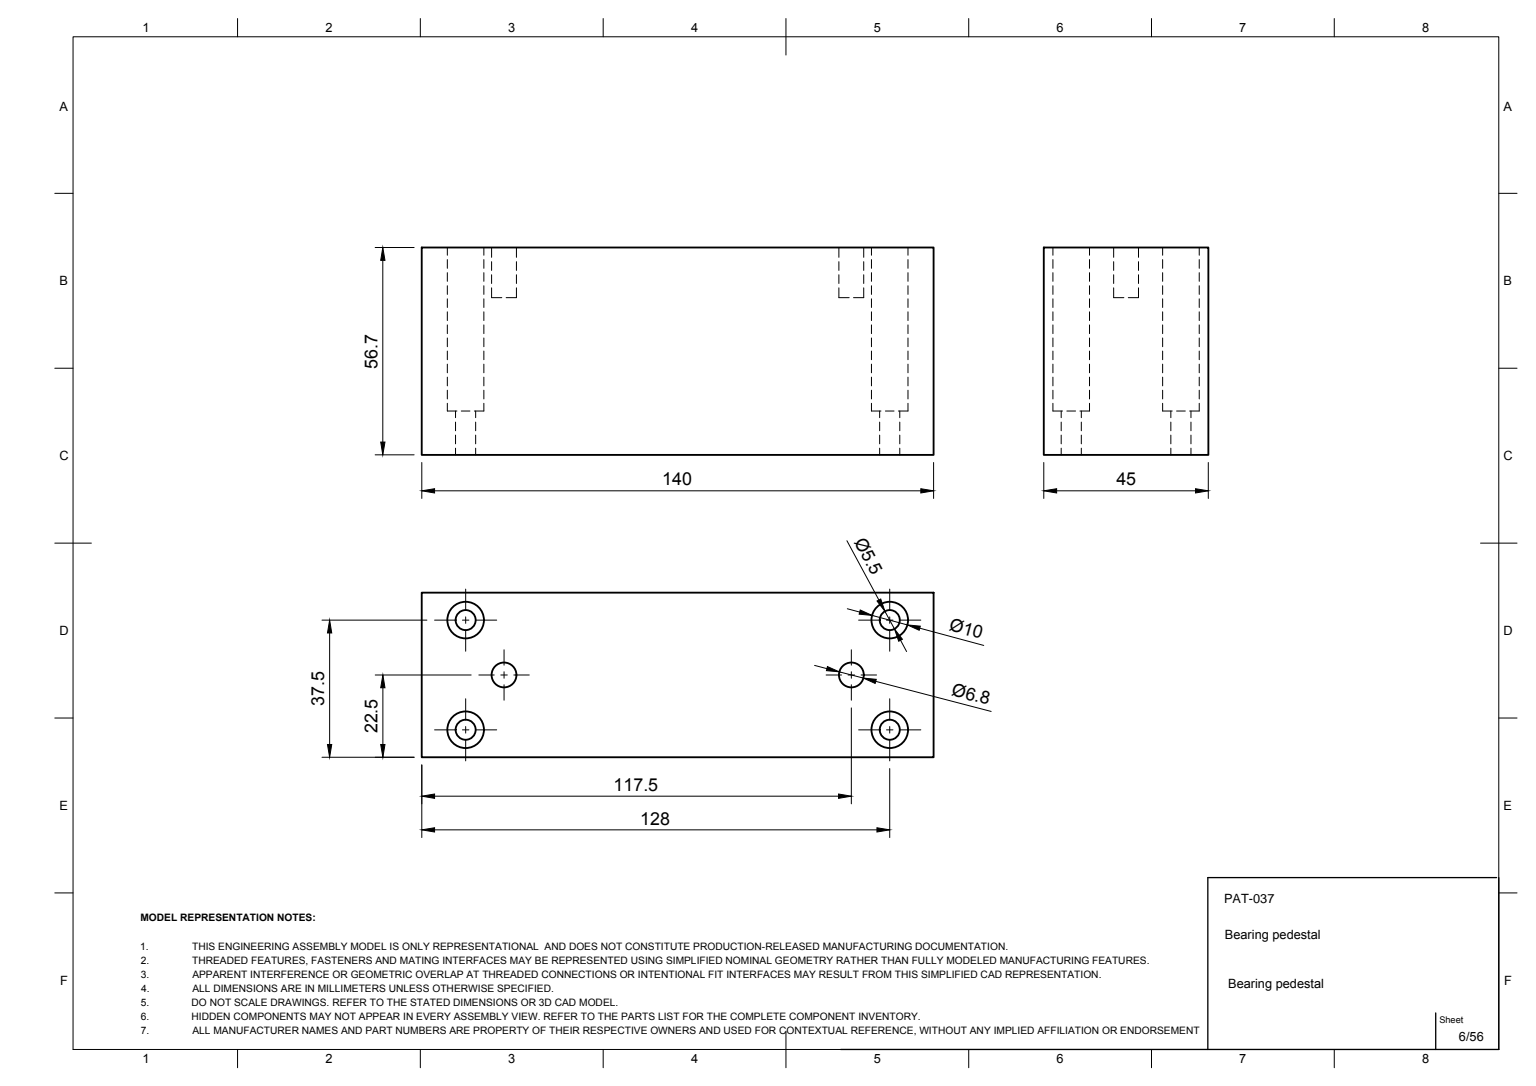
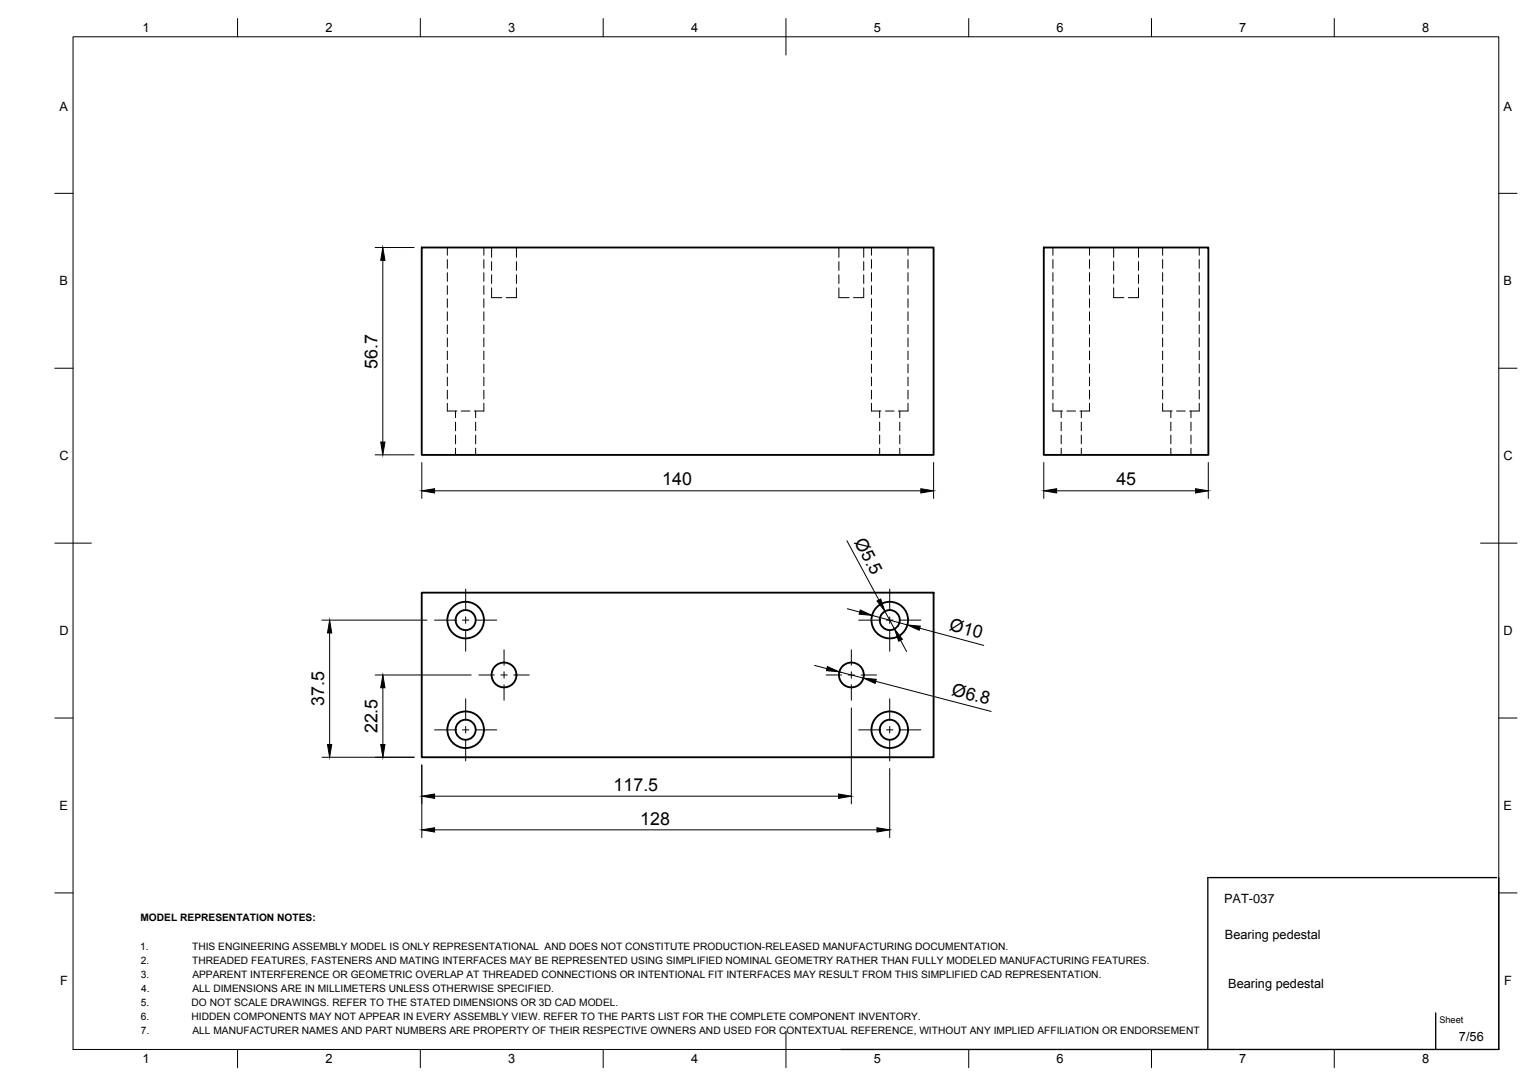
ISO-10303-21;
HEADER;
/* Generated by software containing ST-Developer
 * from STEP Tools, Inc. (www.steptools.com) 
 */

FILE_DESCRIPTION(
/* description */ ('Flywheel Crank-Slider'),
/* implementation_level */ '2;1');

FILE_NAME(
/* name */ 'Bearing pedestal.step',
/* time_stamp */ '2026-10-28T03:23:13-07:00',
/* author */ (''),
/* organization */ (''),
/* preprocessor_version */ 'ST-DEVELOPER v20.2',
/* originating_system */ 'Autodesk Translation Framework v15.17.0.0',
/* authorisation */ '');

FILE_SCHEMA (('AUTOMOTIVE_DESIGN { 1 0 10303 214 3 1 1 }'));
ENDSEC;

DATA;
#10=MECHANICAL_DESIGN_GEOMETRIC_PRESENTATION_REPRESENTATION('',(#669),#17322);
#565=SHAPE_REPRESENTATION_RELATIONSHIP('SRR','None',#17561,#617);
#617=ADVANCED_BREP_SHAPE_REPRESENTATION('',(#730),#17265);
#669=STYLED_ITEM('',(#17931),#730);
#730=MANIFOLD_SOLID_BREP('Body1',#9047);
#809=FACE_BOUND('',#1903,.T.);
#810=FACE_BOUND('',#1906,.T.);
#811=FACE_BOUND('',#1909,.T.);
#812=FACE_BOUND('',#1912,.T.);
#813=FACE_BOUND('',#1922,.T.);
#814=FACE_BOUND('',#1923,.T.);
#815=FACE_BOUND('',#1924,.T.);
#816=FACE_BOUND('',#1925,.T.);
#817=FACE_BOUND('',#1926,.T.);
#818=FACE_BOUND('',#1927,.T.);
#819=FACE_BOUND('',#1929,.T.);
#820=FACE_BOUND('',#1930,.T.);
#821=FACE_BOUND('',#1931,.T.);
#822=FACE_BOUND('',#1932,.T.);
#1017=PLANE('',#9734);
#1018=PLANE('',#9738);
#1019=PLANE('',#9742);
#1020=PLANE('',#9747);
#1021=PLANE('',#9752);
#1022=PLANE('',#9757);
#1023=PLANE('',#9767);
#1024=PLANE('',#9768);
#1025=PLANE('',#9769);
#1026=PLANE('',#9770);
#1027=PLANE('',#9771);
#1028=PLANE('',#9772);
#1338=FACE_OUTER_BOUND('',#1897,.T.);
#1339=FACE_OUTER_BOUND('',#1898,.T.);
#1340=FACE_OUTER_BOUND('',#1899,.T.);
#1341=FACE_OUTER_BOUND('',#1900,.T.);
#1342=FACE_OUTER_BOUND('',#1901,.T.);
#1343=FACE_OUTER_BOUND('',#1902,.T.);
#1344=FACE_OUTER_BOUND('',#1904,.T.);
#1345=FACE_OUTER_BOUND('',#1905,.T.);
#1346=FACE_OUTER_BOUND('',#1907,.T.);
#1347=FACE_OUTER_BOUND('',#1908,.T.);
#1348=FACE_OUTER_BOUND('',#1910,.T.);
#1349=FACE_OUTER_BOUND('',#1911,.T.);
#1350=FACE_OUTER_BOUND('',#1913,.T.);
#1351=FACE_OUTER_BOUND('',#1914,.T.);
#1352=FACE_OUTER_BOUND('',#1915,.T.);
#1353=FACE_OUTER_BOUND('',#1916,.T.);
#1354=FACE_OUTER_BOUND('',#1917,.T.);
#1355=FACE_OUTER_BOUND('',#1918,.T.);
#1356=FACE_OUTER_BOUND('',#1919,.T.);
#1357=FACE_OUTER_BOUND('',#1920,.T.);
#1358=FACE_OUTER_BOUND('',#1921,.T.);
#1359=FACE_OUTER_BOUND('',#1928,.T.);
#1897=EDGE_LOOP('',(#6218,#6219,#6220,#6221));
#1898=EDGE_LOOP('',(#6222));
#1899=EDGE_LOOP('',(#6223,#6224,#6225,#6226));
#1900=EDGE_LOOP('',(#6227));
#1901=EDGE_LOOP('',(#6228,#6229,#6230,#6231));
#1902=EDGE_LOOP('',(#6232));
#1903=EDGE_LOOP('',(#6233));
#1904=EDGE_LOOP('',(#6234,#6235,#6236,#6237));
#1905=EDGE_LOOP('',(#6238));
#1906=EDGE_LOOP('',(#6239));
#1907=EDGE_LOOP('',(#6240,#6241,#6242,#6243));
#1908=EDGE_LOOP('',(#6244));
#1909=EDGE_LOOP('',(#6245));
#1910=EDGE_LOOP('',(#6246,#6247,#6248,#6249));
#1911=EDGE_LOOP('',(#6250));
#1912=EDGE_LOOP('',(#6251));
#1913=EDGE_LOOP('',(#6252,#6253,#6254,#6255));
#1914=EDGE_LOOP('',(#6256,#6257,#6258,#6259));
#1915=EDGE_LOOP('',(#6260,#6261,#6262,#6263));
#1916=EDGE_LOOP('',(#6264,#6265,#6266,#6267));
#1917=EDGE_LOOP('',(#6268,#6269,#6270,#6271));
#1918=EDGE_LOOP('',(#6272,#6273,#6274,#6275));
#1919=EDGE_LOOP('',(#6276,#6277,#6278,#6279));
#1920=EDGE_LOOP('',(#6280,#6281,#6282,#6283));
#1921=EDGE_LOOP('',(#6284,#6285,#6286,#6287));
#1922=EDGE_LOOP('',(#6288));
#1923=EDGE_LOOP('',(#6289));
#1924=EDGE_LOOP('',(#6290));
#1925=EDGE_LOOP('',(#6291));
#1926=EDGE_LOOP('',(#6292));
#1927=EDGE_LOOP('',(#6293));
#1928=EDGE_LOOP('',(#6294,#6295,#6296,#6297));
#1929=EDGE_LOOP('',(#6298));
#1930=EDGE_LOOP('',(#6299));
#1931=EDGE_LOOP('',(#6300));
#1932=EDGE_LOOP('',(#6301));
#2640=LINE('',#13837,#3251);
#2641=LINE('',#13844,#3252);
#2642=LINE('',#13851,#3253);
#2643=LINE('',#13860,#3254);
#2644=LINE('',#13869,#3255);
#2645=LINE('',#13878,#3256);
#2646=LINE('',#13886,#3257);
#2647=LINE('',#13890,#3258);
#2648=LINE('',#13894,#3259);
#2649=LINE('',#13898,#3260);
#2650=LINE('',#13902,#3261);
#2651=LINE('',#13904,#3262);
#2652=LINE('',#13906,#3263);
#2653=LINE('',#13907,#3264);
#2654=LINE('',#13910,#3265);
#2655=LINE('',#13912,#3266);
#2656=LINE('',#13913,#3267);
#2657=LINE('',#13916,#3268);
#2658=LINE('',#13918,#3269);
#2659=LINE('',#13919,#3270);
#2660=LINE('',#13921,#3271);
#2661=LINE('',#13922,#3272);
#3251=VECTOR('',#10950,0.34);
#3252=VECTOR('',#10959,0.34);
#3253=VECTOR('',#10968,0.5);
#3254=VECTOR('',#10979,0.5);
#3255=VECTOR('',#10990,0.5);
#3256=VECTOR('',#11001,0.5);
#3257=VECTOR('',#11012,0.275);
#3258=VECTOR('',#11017,0.275);
#3259=VECTOR('',#11022,0.275);
#3260=VECTOR('',#11027,0.275);
#3261=VECTOR('',#11030,1.);
#3262=VECTOR('',#11031,1.);
#3263=VECTOR('',#11032,1.);
#3264=VECTOR('',#11033,1.);
#3265=VECTOR('',#11036,1.);
#3266=VECTOR('',#11037,1.);
#3267=VECTOR('',#11038,1.);
#3268=VECTOR('',#11041,1.);
#3269=VECTOR('',#11042,1.);
#3270=VECTOR('',#11043,1.);
#3271=VECTOR('',#11046,1.);
#3272=VECTOR('',#11047,1.);
#3862=CIRCLE('',#9732,0.34);
#3863=CIRCLE('',#9733,0.34);
#3864=CIRCLE('',#9736,0.34);
#3865=CIRCLE('',#9737,0.34);
#3866=CIRCLE('',#9740,0.5);
#3867=CIRCLE('',#9741,0.5);
#3868=CIRCLE('',#9743,0.275);
#3869=CIRCLE('',#9745,0.5);
#3870=CIRCLE('',#9746,0.5);
#3871=CIRCLE('',#9748,0.275);
#3872=CIRCLE('',#9750,0.5);
#3873=CIRCLE('',#9751,0.5);
#3874=CIRCLE('',#9753,0.275);
#3875=CIRCLE('',#9755,0.5);
#3876=CIRCLE('',#9756,0.5);
#3877=CIRCLE('',#9758,0.275);
#3878=CIRCLE('',#9760,0.275);
#3879=CIRCLE('',#9762,0.275);
#3880=CIRCLE('',#9764,0.275);
#3881=CIRCLE('',#9766,0.275);
#4309=VERTEX_POINT('',#13834);
#4310=VERTEX_POINT('',#13836);
#4311=VERTEX_POINT('',#13841);
#4312=VERTEX_POINT('',#13843);
#4313=VERTEX_POINT('',#13848);
#4314=VERTEX_POINT('',#13850);
#4315=VERTEX_POINT('',#13854);
#4316=VERTEX_POINT('',#13857);
#4317=VERTEX_POINT('',#13859);
#4318=VERTEX_POINT('',#13863);
#4319=VERTEX_POINT('',#13866);
#4320=VERTEX_POINT('',#13868);
#4321=VERTEX_POINT('',#13872);
#4322=VERTEX_POINT('',#13875);
#4323=VERTEX_POINT('',#13877);
#4324=VERTEX_POINT('',#13881);
#4325=VERTEX_POINT('',#13884);
#4326=VERTEX_POINT('',#13888);
#4327=VERTEX_POINT('',#13892);
#4328=VERTEX_POINT('',#13896);
#4329=VERTEX_POINT('',#13900);
#4330=VERTEX_POINT('',#13901);
#4331=VERTEX_POINT('',#13903);
#4332=VERTEX_POINT('',#13905);
#4333=VERTEX_POINT('',#13909);
#4334=VERTEX_POINT('',#13911);
#4335=VERTEX_POINT('',#13915);
#4336=VERTEX_POINT('',#13917);
#5066=EDGE_CURVE('',#4309,#4309,#3862,.T.);
#5067=EDGE_CURVE('',#4309,#4310,#2640,.T.);
#5068=EDGE_CURVE('',#4310,#4310,#3863,.T.);
#5069=EDGE_CURVE('',#4311,#4311,#3864,.T.);
#5070=EDGE_CURVE('',#4311,#4312,#2641,.T.);
#5071=EDGE_CURVE('',#4312,#4312,#3865,.T.);
#5072=EDGE_CURVE('',#4313,#4313,#3866,.T.);
#5073=EDGE_CURVE('',#4313,#4314,#2642,.T.);
#5074=EDGE_CURVE('',#4314,#4314,#3867,.T.);
#5075=EDGE_CURVE('',#4315,#4315,#3868,.T.);
#5076=EDGE_CURVE('',#4316,#4316,#3869,.T.);
#5077=EDGE_CURVE('',#4316,#4317,#2643,.T.);
#5078=EDGE_CURVE('',#4317,#4317,#3870,.T.);
#5079=EDGE_CURVE('',#4318,#4318,#3871,.T.);
#5080=EDGE_CURVE('',#4319,#4319,#3872,.T.);
#5081=EDGE_CURVE('',#4319,#4320,#2644,.T.);
#5082=EDGE_CURVE('',#4320,#4320,#3873,.T.);
#5083=EDGE_CURVE('',#4321,#4321,#3874,.T.);
#5084=EDGE_CURVE('',#4322,#4322,#3875,.T.);
#5085=EDGE_CURVE('',#4322,#4323,#2645,.T.);
#5086=EDGE_CURVE('',#4323,#4323,#3876,.T.);
#5087=EDGE_CURVE('',#4324,#4324,#3877,.T.);
#5088=EDGE_CURVE('',#4325,#4325,#3878,.T.);
#5089=EDGE_CURVE('',#4325,#4315,#2646,.T.);
#5090=EDGE_CURVE('',#4326,#4326,#3879,.T.);
#5091=EDGE_CURVE('',#4326,#4318,#2647,.T.);
#5092=EDGE_CURVE('',#4327,#4327,#3880,.T.);
#5093=EDGE_CURVE('',#4327,#4321,#2648,.T.);
#5094=EDGE_CURVE('',#4328,#4328,#3881,.T.);
#5095=EDGE_CURVE('',#4328,#4324,#2649,.T.);
#5096=EDGE_CURVE('',#4329,#4330,#2650,.T.);
#5097=EDGE_CURVE('',#4330,#4331,#2651,.T.);
#5098=EDGE_CURVE('',#4332,#4331,#2652,.T.);
#5099=EDGE_CURVE('',#4329,#4332,#2653,.T.);
#5100=EDGE_CURVE('',#4333,#4329,#2654,.T.);
#5101=EDGE_CURVE('',#4334,#4332,#2655,.T.);
#5102=EDGE_CURVE('',#4333,#4334,#2656,.T.);
#5103=EDGE_CURVE('',#4335,#4333,#2657,.T.);
#5104=EDGE_CURVE('',#4336,#4334,#2658,.T.);
#5105=EDGE_CURVE('',#4335,#4336,#2659,.T.);
#5106=EDGE_CURVE('',#4330,#4335,#2660,.T.);
#5107=EDGE_CURVE('',#4331,#4336,#2661,.T.);
#6218=ORIENTED_EDGE('',*,*,#5066,.F.);
#6219=ORIENTED_EDGE('',*,*,#5067,.T.);
#6220=ORIENTED_EDGE('',*,*,#5068,.F.);
#6221=ORIENTED_EDGE('',*,*,#5067,.F.);
#6222=ORIENTED_EDGE('',*,*,#5066,.T.);
#6223=ORIENTED_EDGE('',*,*,#5069,.F.);
#6224=ORIENTED_EDGE('',*,*,#5070,.T.);
#6225=ORIENTED_EDGE('',*,*,#5071,.F.);
#6226=ORIENTED_EDGE('',*,*,#5070,.F.);
#6227=ORIENTED_EDGE('',*,*,#5069,.T.);
#6228=ORIENTED_EDGE('',*,*,#5072,.F.);
#6229=ORIENTED_EDGE('',*,*,#5073,.T.);
#6230=ORIENTED_EDGE('',*,*,#5074,.F.);
#6231=ORIENTED_EDGE('',*,*,#5073,.F.);
#6232=ORIENTED_EDGE('',*,*,#5072,.T.);
#6233=ORIENTED_EDGE('',*,*,#5075,.F.);
#6234=ORIENTED_EDGE('',*,*,#5076,.F.);
#6235=ORIENTED_EDGE('',*,*,#5077,.T.);
#6236=ORIENTED_EDGE('',*,*,#5078,.F.);
#6237=ORIENTED_EDGE('',*,*,#5077,.F.);
#6238=ORIENTED_EDGE('',*,*,#5076,.T.);
#6239=ORIENTED_EDGE('',*,*,#5079,.F.);
#6240=ORIENTED_EDGE('',*,*,#5080,.F.);
#6241=ORIENTED_EDGE('',*,*,#5081,.T.);
#6242=ORIENTED_EDGE('',*,*,#5082,.F.);
#6243=ORIENTED_EDGE('',*,*,#5081,.F.);
#6244=ORIENTED_EDGE('',*,*,#5080,.T.);
#6245=ORIENTED_EDGE('',*,*,#5083,.F.);
#6246=ORIENTED_EDGE('',*,*,#5084,.F.);
#6247=ORIENTED_EDGE('',*,*,#5085,.T.);
#6248=ORIENTED_EDGE('',*,*,#5086,.F.);
#6249=ORIENTED_EDGE('',*,*,#5085,.F.);
#6250=ORIENTED_EDGE('',*,*,#5084,.T.);
#6251=ORIENTED_EDGE('',*,*,#5087,.F.);
#6252=ORIENTED_EDGE('',*,*,#5088,.F.);
#6253=ORIENTED_EDGE('',*,*,#5089,.T.);
#6254=ORIENTED_EDGE('',*,*,#5075,.T.);
#6255=ORIENTED_EDGE('',*,*,#5089,.F.);
#6256=ORIENTED_EDGE('',*,*,#5090,.F.);
#6257=ORIENTED_EDGE('',*,*,#5091,.T.);
#6258=ORIENTED_EDGE('',*,*,#5079,.T.);
#6259=ORIENTED_EDGE('',*,*,#5091,.F.);
#6260=ORIENTED_EDGE('',*,*,#5092,.F.);
#6261=ORIENTED_EDGE('',*,*,#5093,.T.);
#6262=ORIENTED_EDGE('',*,*,#5083,.T.);
#6263=ORIENTED_EDGE('',*,*,#5093,.F.);
#6264=ORIENTED_EDGE('',*,*,#5094,.F.);
#6265=ORIENTED_EDGE('',*,*,#5095,.T.);
#6266=ORIENTED_EDGE('',*,*,#5087,.T.);
#6267=ORIENTED_EDGE('',*,*,#5095,.F.);
#6268=ORIENTED_EDGE('',*,*,#5096,.T.);
#6269=ORIENTED_EDGE('',*,*,#5097,.T.);
#6270=ORIENTED_EDGE('',*,*,#5098,.F.);
#6271=ORIENTED_EDGE('',*,*,#5099,.F.);
#6272=ORIENTED_EDGE('',*,*,#5100,.T.);
#6273=ORIENTED_EDGE('',*,*,#5099,.T.);
#6274=ORIENTED_EDGE('',*,*,#5101,.F.);
#6275=ORIENTED_EDGE('',*,*,#5102,.F.);
#6276=ORIENTED_EDGE('',*,*,#5103,.T.);
#6277=ORIENTED_EDGE('',*,*,#5102,.T.);
#6278=ORIENTED_EDGE('',*,*,#5104,.F.);
#6279=ORIENTED_EDGE('',*,*,#5105,.F.);
#6280=ORIENTED_EDGE('',*,*,#5106,.T.);
#6281=ORIENTED_EDGE('',*,*,#5105,.T.);
#6282=ORIENTED_EDGE('',*,*,#5107,.F.);
#6283=ORIENTED_EDGE('',*,*,#5097,.F.);
#6284=ORIENTED_EDGE('',*,*,#5107,.T.);
#6285=ORIENTED_EDGE('',*,*,#5104,.T.);
#6286=ORIENTED_EDGE('',*,*,#5101,.T.);
#6287=ORIENTED_EDGE('',*,*,#5098,.T.);
#6288=ORIENTED_EDGE('',*,*,#5068,.T.);
#6289=ORIENTED_EDGE('',*,*,#5071,.T.);
#6290=ORIENTED_EDGE('',*,*,#5086,.T.);
#6291=ORIENTED_EDGE('',*,*,#5082,.T.);
#6292=ORIENTED_EDGE('',*,*,#5078,.T.);
#6293=ORIENTED_EDGE('',*,*,#5074,.T.);
#6294=ORIENTED_EDGE('',*,*,#5106,.F.);
#6295=ORIENTED_EDGE('',*,*,#5096,.F.);
#6296=ORIENTED_EDGE('',*,*,#5100,.F.);
#6297=ORIENTED_EDGE('',*,*,#5103,.F.);
#6298=ORIENTED_EDGE('',*,*,#5088,.T.);
#6299=ORIENTED_EDGE('',*,*,#5090,.T.);
#6300=ORIENTED_EDGE('',*,*,#5092,.T.);
#6301=ORIENTED_EDGE('',*,*,#5094,.T.);
#8342=CYLINDRICAL_SURFACE('',#9731,0.34);
#8343=CYLINDRICAL_SURFACE('',#9735,0.34);
#8344=CYLINDRICAL_SURFACE('',#9739,0.5);
#8345=CYLINDRICAL_SURFACE('',#9744,0.5);
#8346=CYLINDRICAL_SURFACE('',#9749,0.5);
#8347=CYLINDRICAL_SURFACE('',#9754,0.5);
#8348=CYLINDRICAL_SURFACE('',#9759,0.275);
#8349=CYLINDRICAL_SURFACE('',#9761,0.275);
#8350=CYLINDRICAL_SURFACE('',#9763,0.275);
#8351=CYLINDRICAL_SURFACE('',#9765,0.275);
#8529=ADVANCED_FACE('',(#1338),#8342,.F.);
#8530=ADVANCED_FACE('',(#1339),#1017,.T.);
#8531=ADVANCED_FACE('',(#1340),#8343,.F.);
#8532=ADVANCED_FACE('',(#1341),#1018,.T.);
#8533=ADVANCED_FACE('',(#1342),#8344,.F.);
#8534=ADVANCED_FACE('',(#1343,#809),#1019,.T.);
#8535=ADVANCED_FACE('',(#1344),#8345,.F.);
#8536=ADVANCED_FACE('',(#1345,#810),#1020,.T.);
#8537=ADVANCED_FACE('',(#1346),#8346,.F.);
#8538=ADVANCED_FACE('',(#1347,#811),#1021,.T.);
#8539=ADVANCED_FACE('',(#1348),#8347,.F.);
#8540=ADVANCED_FACE('',(#1349,#812),#1022,.T.);
#8541=ADVANCED_FACE('',(#1350),#8348,.F.);
#8542=ADVANCED_FACE('',(#1351),#8349,.F.);
#8543=ADVANCED_FACE('',(#1352),#8350,.F.);
#8544=ADVANCED_FACE('',(#1353),#8351,.F.);
#8545=ADVANCED_FACE('',(#1354),#1023,.T.);
#8546=ADVANCED_FACE('',(#1355),#1024,.T.);
#8547=ADVANCED_FACE('',(#1356),#1025,.T.);
#8548=ADVANCED_FACE('',(#1357),#1026,.T.);
#8549=ADVANCED_FACE('',(#1358,#813,#814,#815,#816,#817,#818),#1027,.T.);
#8550=ADVANCED_FACE('',(#1359,#819,#820,#821,#822),#1028,.F.);
#9047=CLOSED_SHELL('',(#8529,#8530,#8531,#8532,#8533,#8534,#8535,#8536,
#8537,#8538,#8539,#8540,#8541,#8542,#8543,#8544,#8545,#8546,#8547,#8548,
#8549,#8550));
#9730=AXIS2_PLACEMENT_3D('',#13832,#10944,#10945);
#9731=AXIS2_PLACEMENT_3D('',#13833,#10946,#10947);
#9732=AXIS2_PLACEMENT_3D('',#13835,#10948,#10949);
#9733=AXIS2_PLACEMENT_3D('',#13838,#10951,#10952);
#9734=AXIS2_PLACEMENT_3D('',#13839,#10953,#10954);
#9735=AXIS2_PLACEMENT_3D('',#13840,#10955,#10956);
#9736=AXIS2_PLACEMENT_3D('',#13842,#10957,#10958);
#9737=AXIS2_PLACEMENT_3D('',#13845,#10960,#10961);
#9738=AXIS2_PLACEMENT_3D('',#13846,#10962,#10963);
#9739=AXIS2_PLACEMENT_3D('',#13847,#10964,#10965);
#9740=AXIS2_PLACEMENT_3D('',#13849,#10966,#10967);
#9741=AXIS2_PLACEMENT_3D('',#13852,#10969,#10970);
#9742=AXIS2_PLACEMENT_3D('',#13853,#10971,#10972);
#9743=AXIS2_PLACEMENT_3D('',#13855,#10973,#10974);
#9744=AXIS2_PLACEMENT_3D('',#13856,#10975,#10976);
#9745=AXIS2_PLACEMENT_3D('',#13858,#10977,#10978);
#9746=AXIS2_PLACEMENT_3D('',#13861,#10980,#10981);
#9747=AXIS2_PLACEMENT_3D('',#13862,#10982,#10983);
#9748=AXIS2_PLACEMENT_3D('',#13864,#10984,#10985);
#9749=AXIS2_PLACEMENT_3D('',#13865,#10986,#10987);
#9750=AXIS2_PLACEMENT_3D('',#13867,#10988,#10989);
#9751=AXIS2_PLACEMENT_3D('',#13870,#10991,#10992);
#9752=AXIS2_PLACEMENT_3D('',#13871,#10993,#10994);
#9753=AXIS2_PLACEMENT_3D('',#13873,#10995,#10996);
#9754=AXIS2_PLACEMENT_3D('',#13874,#10997,#10998);
#9755=AXIS2_PLACEMENT_3D('',#13876,#10999,#11000);
#9756=AXIS2_PLACEMENT_3D('',#13879,#11002,#11003);
#9757=AXIS2_PLACEMENT_3D('',#13880,#11004,#11005);
#9758=AXIS2_PLACEMENT_3D('',#13882,#11006,#11007);
#9759=AXIS2_PLACEMENT_3D('',#13883,#11008,#11009);
#9760=AXIS2_PLACEMENT_3D('',#13885,#11010,#11011);
#9761=AXIS2_PLACEMENT_3D('',#13887,#11013,#11014);
#9762=AXIS2_PLACEMENT_3D('',#13889,#11015,#11016);
#9763=AXIS2_PLACEMENT_3D('',#13891,#11018,#11019);
#9764=AXIS2_PLACEMENT_3D('',#13893,#11020,#11021);
#9765=AXIS2_PLACEMENT_3D('',#13895,#11023,#11024);
#9766=AXIS2_PLACEMENT_3D('',#13897,#11025,#11026);
#9767=AXIS2_PLACEMENT_3D('',#13899,#11028,#11029);
#9768=AXIS2_PLACEMENT_3D('',#13908,#11034,#11035);
#9769=AXIS2_PLACEMENT_3D('',#13914,#11039,#11040);
#9770=AXIS2_PLACEMENT_3D('',#13920,#11044,#11045);
#9771=AXIS2_PLACEMENT_3D('',#13923,#11048,#11049);
#9772=AXIS2_PLACEMENT_3D('',#13924,#11050,#11051);
#10944=DIRECTION('axis',(0.,0.,1.));
#10945=DIRECTION('refdir',(1.,0.,0.));
#10946=DIRECTION('center_axis',(0.,0.,1.));
#10947=DIRECTION('ref_axis',(1.,0.,0.));
#10948=DIRECTION('center_axis',(0.,0.,1.));
#10949=DIRECTION('ref_axis',(1.,0.,0.));
#10950=DIRECTION('',(0.,0.,1.));
#10951=DIRECTION('center_axis',(0.,0.,-1.));
#10952=DIRECTION('ref_axis',(1.,0.,0.));
#10953=DIRECTION('center_axis',(0.,0.,1.));
#10954=DIRECTION('ref_axis',(1.,0.,0.));
#10955=DIRECTION('center_axis',(0.,0.,1.));
#10956=DIRECTION('ref_axis',(1.,0.,0.));
#10957=DIRECTION('center_axis',(0.,0.,1.));
#10958=DIRECTION('ref_axis',(1.,0.,0.));
#10959=DIRECTION('',(0.,0.,1.));
#10960=DIRECTION('center_axis',(0.,0.,-1.));
#10961=DIRECTION('ref_axis',(1.,0.,0.));
#10962=DIRECTION('center_axis',(0.,0.,1.));
#10963=DIRECTION('ref_axis',(1.,0.,0.));
#10964=DIRECTION('center_axis',(0.,0.,1.));
#10965=DIRECTION('ref_axis',(1.,0.,0.));
#10966=DIRECTION('center_axis',(0.,0.,1.));
#10967=DIRECTION('ref_axis',(1.,0.,0.));
#10968=DIRECTION('',(0.,0.,1.));
#10969=DIRECTION('center_axis',(0.,0.,-1.));
#10970=DIRECTION('ref_axis',(1.,0.,0.));
#10971=DIRECTION('center_axis',(0.,0.,1.));
#10972=DIRECTION('ref_axis',(1.,0.,0.));
#10973=DIRECTION('center_axis',(0.,0.,1.));
#10974=DIRECTION('ref_axis',(1.,0.,0.));
#10975=DIRECTION('center_axis',(0.,0.,1.));
#10976=DIRECTION('ref_axis',(1.,0.,0.));
#10977=DIRECTION('center_axis',(0.,0.,1.));
#10978=DIRECTION('ref_axis',(1.,0.,0.));
#10979=DIRECTION('',(0.,0.,1.));
#10980=DIRECTION('center_axis',(0.,0.,-1.));
#10981=DIRECTION('ref_axis',(1.,0.,0.));
#10982=DIRECTION('center_axis',(0.,0.,1.));
#10983=DIRECTION('ref_axis',(1.,0.,0.));
#10984=DIRECTION('center_axis',(0.,0.,1.));
#10985=DIRECTION('ref_axis',(1.,0.,0.));
#10986=DIRECTION('center_axis',(0.,0.,1.));
#10987=DIRECTION('ref_axis',(1.,0.,0.));
#10988=DIRECTION('center_axis',(0.,0.,1.));
#10989=DIRECTION('ref_axis',(1.,0.,0.));
#10990=DIRECTION('',(0.,0.,1.));
#10991=DIRECTION('center_axis',(0.,0.,-1.));
#10992=DIRECTION('ref_axis',(1.,0.,0.));
#10993=DIRECTION('center_axis',(0.,0.,1.));
#10994=DIRECTION('ref_axis',(1.,0.,0.));
#10995=DIRECTION('center_axis',(0.,0.,1.));
#10996=DIRECTION('ref_axis',(1.,0.,0.));
#10997=DIRECTION('center_axis',(0.,0.,1.));
#10998=DIRECTION('ref_axis',(1.,0.,0.));
#10999=DIRECTION('center_axis',(0.,0.,1.));
#11000=DIRECTION('ref_axis',(1.,0.,0.));
#11001=DIRECTION('',(0.,0.,1.));
#11002=DIRECTION('center_axis',(0.,0.,-1.));
#11003=DIRECTION('ref_axis',(1.,0.,0.));
#11004=DIRECTION('center_axis',(0.,0.,1.));
#11005=DIRECTION('ref_axis',(1.,0.,0.));
#11006=DIRECTION('center_axis',(0.,0.,1.));
#11007=DIRECTION('ref_axis',(1.,0.,0.));
#11008=DIRECTION('center_axis',(0.,0.,1.));
#11009=DIRECTION('ref_axis',(1.,0.,0.));
#11010=DIRECTION('center_axis',(0.,0.,1.));
#11011=DIRECTION('ref_axis',(1.,0.,0.));
#11012=DIRECTION('',(0.,0.,1.));
#11013=DIRECTION('center_axis',(0.,0.,1.));
#11014=DIRECTION('ref_axis',(1.,0.,0.));
#11015=DIRECTION('center_axis',(0.,0.,1.));
#11016=DIRECTION('ref_axis',(1.,0.,0.));
#11017=DIRECTION('',(0.,0.,1.));
#11018=DIRECTION('center_axis',(0.,0.,1.));
#11019=DIRECTION('ref_axis',(1.,0.,0.));
#11020=DIRECTION('center_axis',(0.,0.,1.));
#11021=DIRECTION('ref_axis',(1.,0.,0.));
#11022=DIRECTION('',(0.,0.,1.));
#11023=DIRECTION('center_axis',(0.,0.,1.));
#11024=DIRECTION('ref_axis',(1.,0.,0.));
#11025=DIRECTION('center_axis',(0.,0.,1.));
#11026=DIRECTION('ref_axis',(1.,0.,0.));
#11027=DIRECTION('',(0.,0.,1.));
#11028=DIRECTION('center_axis',(0.,1.,0.));
#11029=DIRECTION('ref_axis',(-1.,0.,0.));
#11030=DIRECTION('',(-1.,0.,0.));
#11031=DIRECTION('',(0.,0.,1.));
#11032=DIRECTION('',(-1.,0.,0.));
#11033=DIRECTION('',(0.,0.,1.));
#11034=DIRECTION('center_axis',(1.,0.,0.));
#11035=DIRECTION('ref_axis',(0.,1.,0.));
#11036=DIRECTION('',(0.,1.,0.));
#11037=DIRECTION('',(0.,1.,0.));
#11038=DIRECTION('',(0.,0.,1.));
#11039=DIRECTION('center_axis',(0.,-1.,0.));
#11040=DIRECTION('ref_axis',(1.,0.,0.));
#11041=DIRECTION('',(1.,0.,0.));
#11042=DIRECTION('',(1.,0.,0.));
#11043=DIRECTION('',(0.,0.,1.));
#11044=DIRECTION('center_axis',(-1.,0.,0.));
#11045=DIRECTION('ref_axis',(0.,-1.,0.));
#11046=DIRECTION('',(0.,-1.,0.));
#11047=DIRECTION('',(0.,-1.,0.));
#11048=DIRECTION('center_axis',(0.,0.,1.));
#11049=DIRECTION('ref_axis',(1.,0.,0.));
#11050=DIRECTION('center_axis',(0.,0.,1.));
#11051=DIRECTION('ref_axis',(1.,0.,0.));
#13832=CARTESIAN_POINT('',(0.,0.,0.));
#13833=CARTESIAN_POINT('Origin',(-4.75,-15.,5.3));
#13834=CARTESIAN_POINT('',(-5.09,-15.,5.3));
#13835=CARTESIAN_POINT('Origin',(-4.75,-15.,5.3));
#13836=CARTESIAN_POINT('',(-5.09,-15.,6.67));
#13837=CARTESIAN_POINT('',(-5.09,-15.,5.3));
#13838=CARTESIAN_POINT('Origin',(-4.75,-15.,6.67));
#13839=CARTESIAN_POINT('Origin',(-4.75,-15.,5.3));
#13840=CARTESIAN_POINT('Origin',(4.75,-15.,5.3));
#13841=CARTESIAN_POINT('',(4.41,-15.,5.3));
#13842=CARTESIAN_POINT('Origin',(4.75,-15.,5.3));
#13843=CARTESIAN_POINT('',(4.41,-15.,6.67));
#13844=CARTESIAN_POINT('',(4.41,-15.,5.3));
#13845=CARTESIAN_POINT('Origin',(4.75,-15.,6.67));
#13846=CARTESIAN_POINT('Origin',(4.75,-15.,5.3));
#13847=CARTESIAN_POINT('Origin',(5.8,-16.5,2.2));
#13848=CARTESIAN_POINT('',(5.3,-16.5,2.2));
#13849=CARTESIAN_POINT('Origin',(5.8,-16.5,2.2));
#13850=CARTESIAN_POINT('',(5.3,-16.5,6.67));
#13851=CARTESIAN_POINT('',(5.3,-16.5,2.2));
#13852=CARTESIAN_POINT('Origin',(5.8,-16.5,6.67));
#13853=CARTESIAN_POINT('Origin',(5.8,-16.5,2.2));
#13854=CARTESIAN_POINT('',(5.525,-16.5,2.2));
#13855=CARTESIAN_POINT('Origin',(5.8,-16.5,2.2));
#13856=CARTESIAN_POINT('Origin',(-5.8,-13.5,2.2));
#13857=CARTESIAN_POINT('',(-6.3,-13.5,2.2));
#13858=CARTESIAN_POINT('Origin',(-5.8,-13.5,2.2));
#13859=CARTESIAN_POINT('',(-6.3,-13.5,6.67));
#13860=CARTESIAN_POINT('',(-6.3,-13.5,2.2));
#13861=CARTESIAN_POINT('Origin',(-5.8,-13.5,6.67));
#13862=CARTESIAN_POINT('Origin',(-5.8,-13.5,2.2));
#13863=CARTESIAN_POINT('',(-6.075,-13.5,2.2));
#13864=CARTESIAN_POINT('Origin',(-5.8,-13.5,2.2));
#13865=CARTESIAN_POINT('Origin',(-5.8,-16.5,2.2));
#13866=CARTESIAN_POINT('',(-6.3,-16.5,2.2));
#13867=CARTESIAN_POINT('Origin',(-5.8,-16.5,2.2));
#13868=CARTESIAN_POINT('',(-6.3,-16.5,6.67));
#13869=CARTESIAN_POINT('',(-6.3,-16.5,2.2));
#13870=CARTESIAN_POINT('Origin',(-5.8,-16.5,6.67));
#13871=CARTESIAN_POINT('Origin',(-5.8,-16.5,2.2));
#13872=CARTESIAN_POINT('',(-6.075,-16.5,2.2));
#13873=CARTESIAN_POINT('Origin',(-5.8,-16.5,2.2));
#13874=CARTESIAN_POINT('Origin',(5.8,-13.5,2.2));
#13875=CARTESIAN_POINT('',(5.3,-13.5,2.2));
#13876=CARTESIAN_POINT('Origin',(5.8,-13.5,2.2));
#13877=CARTESIAN_POINT('',(5.3,-13.5,6.67));
#13878=CARTESIAN_POINT('',(5.3,-13.5,2.2));
#13879=CARTESIAN_POINT('Origin',(5.8,-13.5,6.67));
#13880=CARTESIAN_POINT('Origin',(5.8,-13.5,2.2));
#13881=CARTESIAN_POINT('',(5.525,-13.5,2.2));
#13882=CARTESIAN_POINT('Origin',(5.8,-13.5,2.2));
#13883=CARTESIAN_POINT('Origin',(5.8,-16.5,0.9));
#13884=CARTESIAN_POINT('',(5.525,-16.5,1.));
#13885=CARTESIAN_POINT('Origin',(5.8,-16.5,1.));
#13886=CARTESIAN_POINT('',(5.525,-16.5,0.9));
#13887=CARTESIAN_POINT('Origin',(-5.8,-13.5,0.9));
#13888=CARTESIAN_POINT('',(-6.075,-13.5,1.));
#13889=CARTESIAN_POINT('Origin',(-5.8,-13.5,1.));
#13890=CARTESIAN_POINT('',(-6.075,-13.5,0.9));
#13891=CARTESIAN_POINT('Origin',(-5.8,-16.5,0.9));
#13892=CARTESIAN_POINT('',(-6.075,-16.5,1.));
#13893=CARTESIAN_POINT('Origin',(-5.8,-16.5,1.));
#13894=CARTESIAN_POINT('',(-6.075,-16.5,0.9));
#13895=CARTESIAN_POINT('Origin',(5.8,-13.5,0.9));
#13896=CARTESIAN_POINT('',(5.525,-13.5,1.));
#13897=CARTESIAN_POINT('Origin',(5.8,-13.5,1.));
#13898=CARTESIAN_POINT('',(5.525,-13.5,0.9));
#13899=CARTESIAN_POINT('Origin',(7.,-12.75,1.));
#13900=CARTESIAN_POINT('',(7.,-12.75,1.));
#13901=CARTESIAN_POINT('',(-7.,-12.75,1.));
#13902=CARTESIAN_POINT('',(7.,-12.75,1.));
#13903=CARTESIAN_POINT('',(-7.,-12.75,6.67));
#13904=CARTESIAN_POINT('',(-7.,-12.75,1.));
#13905=CARTESIAN_POINT('',(7.,-12.75,6.67));
#13906=CARTESIAN_POINT('',(7.,-12.75,6.67));
#13907=CARTESIAN_POINT('',(7.,-12.75,1.));
#13908=CARTESIAN_POINT('Origin',(7.,-17.25,1.));
#13909=CARTESIAN_POINT('',(7.,-17.25,1.));
#13910=CARTESIAN_POINT('',(7.,-17.25,1.));
#13911=CARTESIAN_POINT('',(7.,-17.25,6.67));
#13912=CARTESIAN_POINT('',(7.,-17.25,6.67));
#13913=CARTESIAN_POINT('',(7.,-17.25,1.));
#13914=CARTESIAN_POINT('Origin',(-7.,-17.25,1.));
#13915=CARTESIAN_POINT('',(-7.,-17.25,1.));
#13916=CARTESIAN_POINT('',(-7.,-17.25,1.));
#13917=CARTESIAN_POINT('',(-7.,-17.25,6.67));
#13918=CARTESIAN_POINT('',(-7.,-17.25,6.67));
#13919=CARTESIAN_POINT('',(-7.,-17.25,1.));
#13920=CARTESIAN_POINT('Origin',(-7.,-12.75,1.));
#13921=CARTESIAN_POINT('',(-7.,-12.75,1.));
#13922=CARTESIAN_POINT('',(-7.,-12.75,6.67));
#13923=CARTESIAN_POINT('Origin',(0.,-15.,6.67));
#13924=CARTESIAN_POINT('Origin',(0.,-15.,1.));
#17204=UNCERTAINTY_MEASURE_WITH_UNIT(LENGTH_MEASURE(0.001),#17323,
'DISTANCE_ACCURACY_VALUE',
'Maximum model space distance between geometric entities at asserted c
onnectivities');
#17261=UNCERTAINTY_MEASURE_WITH_UNIT(LENGTH_MEASURE(0.001),#17323,
'DISTANCE_ACCURACY_VALUE',
'Maximum model space distance between geometric entities at asserted c
onnectivities');
#17265=(
GEOMETRIC_REPRESENTATION_CONTEXT(3)
GLOBAL_UNCERTAINTY_ASSIGNED_CONTEXT((#17204))
GLOBAL_UNIT_ASSIGNED_CONTEXT((#17323,#17325,#17326))
REPRESENTATION_CONTEXT('','3D')
);
#17322=(
GEOMETRIC_REPRESENTATION_CONTEXT(3)
GLOBAL_UNCERTAINTY_ASSIGNED_CONTEXT((#17261))
GLOBAL_UNIT_ASSIGNED_CONTEXT((#17323,#17325,#17326))
REPRESENTATION_CONTEXT('','3D')
);
#17323=(
LENGTH_UNIT()
NAMED_UNIT(*)
SI_UNIT(.CENTI.,.METRE.)
);
#17325=(
NAMED_UNIT(*)
PLANE_ANGLE_UNIT()
SI_UNIT($,.RADIAN.)
);
#17326=(
NAMED_UNIT(*)
SI_UNIT($,.STERADIAN.)
SOLID_ANGLE_UNIT()
);
#17330=SHAPE_DEFINITION_REPRESENTATION(#17390,#17561);
#17390=PRODUCT_DEFINITION_SHAPE('',$,#17622);
#17561=SHAPE_REPRESENTATION('',(#9730),#17265);
#17618=PRODUCT_DEFINITION_CONTEXT('part definition',#17800,'design');
#17622=PRODUCT_DEFINITION('Bearing pedestal','Bearing pedestal',#17682,
#17618);
#17682=PRODUCT_DEFINITION_FORMATION('',$,#17805);
#17800=APPLICATION_CONTEXT(
'Core Data for Automotive Mechanical Design Process');
#17801=PRODUCT_CONTEXT('part definition',#17800,'mechanical');
#17805=PRODUCT('Bearing pedestal','Bearing pedestal','Bearing pedestal',
(#17801));
#17925=COLOUR_RGB('Grey',0.48,0.52,0.57);
#17926=FILL_AREA_STYLE_COLOUR('',#17925);
#17927=FILL_AREA_STYLE('',(#17926));
#17928=SURFACE_STYLE_FILL_AREA(#17927);
#17929=SURFACE_SIDE_STYLE('',(#17928));
#17930=SURFACE_STYLE_USAGE(.BOTH.,#17929);
#17931=PRESENTATION_STYLE_ASSIGNMENT((#17930));
ENDSEC;
END-ISO-10303-21;
